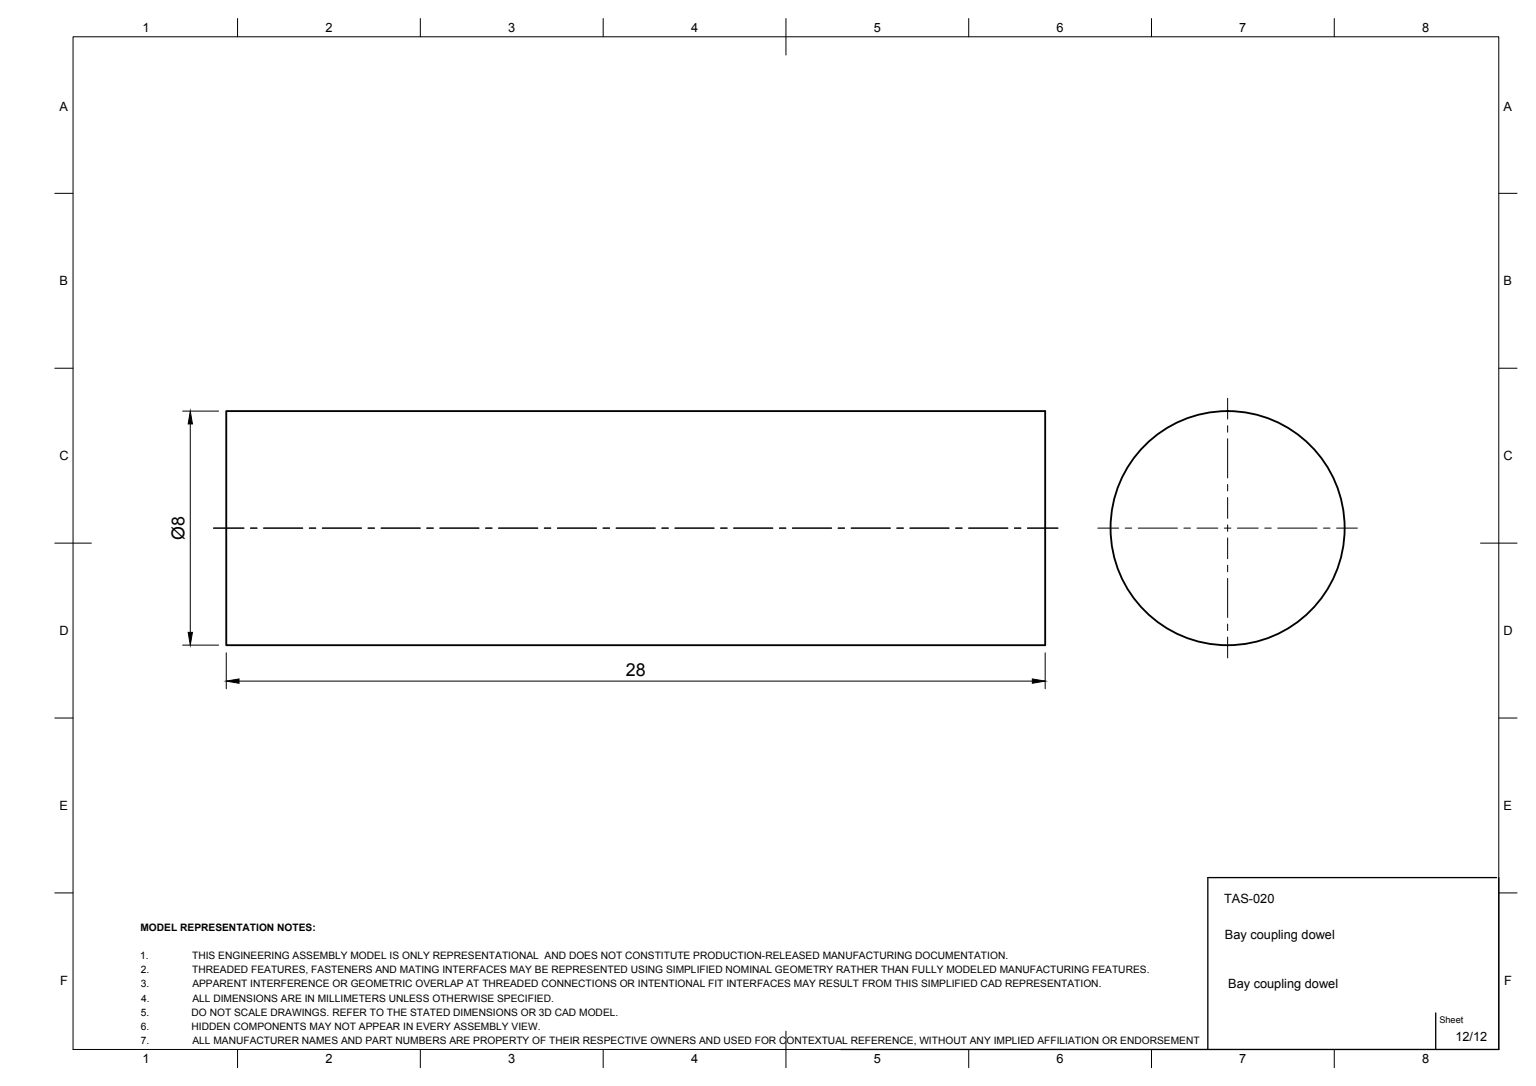
ISO-10303-21;
HEADER;
/* Generated by software containing ST-Developer
 * from STEP Tools, Inc. (www.steptools.com) 
 */

FILE_DESCRIPTION(
/* description */ (''),
/* implementation_level */ '2;1');

FILE_NAME(
/* name */ 'Bay coupling dowel.step',
/* time_stamp */ '2026-11-15T17:46:57-08:00',
/* author */ (''),
/* organization */ (''),
/* preprocessor_version */ 'ST-DEVELOPER v20.2',
/* originating_system */ 'Autodesk Translation Framework v15.17.0.0',
/* authorisation */ '');

FILE_SCHEMA (('AUTOMOTIVE_DESIGN { 1 0 10303 214 3 1 1 }'));
ENDSEC;

DATA;
#10=MECHANICAL_DESIGN_GEOMETRIC_PRESENTATION_REPRESENTATION('',(#386),#12963);
#362=SHAPE_REPRESENTATION_RELATIONSHIP('SRR','None',#13046,#374);
#374=ADVANCED_BREP_SHAPE_REPRESENTATION('',(#398),#12962);
#386=STYLED_ITEM('',(#13115),#398);
#398=MANIFOLD_SOLID_BREP('Body1',#4820);
#570=PLANE('',#5299);
#571=PLANE('',#5300);
#825=FACE_OUTER_BOUND('',#1123,.T.);
#826=FACE_OUTER_BOUND('',#1124,.T.);
#827=FACE_OUTER_BOUND('',#1125,.T.);
#1123=EDGE_LOOP('',(#4426,#4427,#4428,#4429));
#1124=EDGE_LOOP('',(#4430));
#1125=EDGE_LOOP('',(#4431));
#1527=LINE('',#12892,#1929);
#1929=VECTOR('',#6430,0.4);
#2010=CIRCLE('',#5297,0.4);
#2011=CIRCLE('',#5298,0.4);
#2450=VERTEX_POINT('',#12889);
#2451=VERTEX_POINT('',#12891);
#3109=EDGE_CURVE('',#2450,#2450,#2010,.T.);
#3110=EDGE_CURVE('',#2450,#2451,#1527,.T.);
#3111=EDGE_CURVE('',#2451,#2451,#2011,.T.);
#4426=ORIENTED_EDGE('',*,*,#3109,.F.);
#4427=ORIENTED_EDGE('',*,*,#3110,.T.);
#4428=ORIENTED_EDGE('',*,*,#3111,.T.);
#4429=ORIENTED_EDGE('',*,*,#3110,.F.);
#4430=ORIENTED_EDGE('',*,*,#3109,.T.);
#4431=ORIENTED_EDGE('',*,*,#3111,.F.);
#4552=CYLINDRICAL_SURFACE('',#5296,0.4);
#4806=ADVANCED_FACE('',(#825),#4552,.T.);
#4807=ADVANCED_FACE('',(#826),#570,.T.);
#4808=ADVANCED_FACE('',(#827),#571,.F.);
#4820=CLOSED_SHELL('',(#4806,#4807,#4808));
#5295=AXIS2_PLACEMENT_3D('',#12887,#6424,#6425);
#5296=AXIS2_PLACEMENT_3D('',#12888,#6426,#6427);
#5297=AXIS2_PLACEMENT_3D('',#12890,#6428,#6429);
#5298=AXIS2_PLACEMENT_3D('',#12893,#6431,#6432);
#5299=AXIS2_PLACEMENT_3D('',#12894,#6433,#6434);
#5300=AXIS2_PLACEMENT_3D('',#12895,#6435,#6436);
#6424=DIRECTION('axis',(0.,0.,1.));
#6425=DIRECTION('refdir',(1.,0.,0.));
#6426=DIRECTION('center_axis',(0.,0.,1.));
#6427=DIRECTION('ref_axis',(1.,0.,0.));
#6428=DIRECTION('center_axis',(0.,0.,1.));
#6429=DIRECTION('ref_axis',(1.,0.,0.));
#6430=DIRECTION('',(0.,0.,-1.));
#6431=DIRECTION('center_axis',(0.,0.,1.));
#6432=DIRECTION('ref_axis',(1.,0.,0.));
#6433=DIRECTION('center_axis',(0.,0.,1.));
#6434=DIRECTION('ref_axis',(1.,0.,0.));
#6435=DIRECTION('center_axis',(0.,0.,1.));
#6436=DIRECTION('ref_axis',(1.,0.,0.));
#12887=CARTESIAN_POINT('',(0.,0.,0.));
#12888=CARTESIAN_POINT('Origin',(0.,0.,0.));
#12889=CARTESIAN_POINT('',(-0.4,-4.89858719658941E-17,2.8));
#12890=CARTESIAN_POINT('Origin',(0.,0.,2.8));
#12891=CARTESIAN_POINT('',(-0.4,-4.89858719658941E-17,0.));
#12892=CARTESIAN_POINT('',(-0.4,-4.89858719658941E-17,0.));
#12893=CARTESIAN_POINT('Origin',(0.,0.,0.));
#12894=CARTESIAN_POINT('Origin',(0.,0.,2.8));
#12895=CARTESIAN_POINT('Origin',(0.,0.,0.));
#12948=UNCERTAINTY_MEASURE_WITH_UNIT(LENGTH_MEASURE(0.001),#12964,
'DISTANCE_ACCURACY_VALUE',
'Maximum model space distance between geometric entities at asserted c
onnectivities');
#12949=UNCERTAINTY_MEASURE_WITH_UNIT(LENGTH_MEASURE(0.001),#12964,
'DISTANCE_ACCURACY_VALUE',
'Maximum model space distance between geometric entities at asserted c
onnectivities');
#12962=(
GEOMETRIC_REPRESENTATION_CONTEXT(3)
GLOBAL_UNCERTAINTY_ASSIGNED_CONTEXT((#12948))
GLOBAL_UNIT_ASSIGNED_CONTEXT((#12964,#12966,#12967))
REPRESENTATION_CONTEXT('','3D')
);
#12963=(
GEOMETRIC_REPRESENTATION_CONTEXT(3)
GLOBAL_UNCERTAINTY_ASSIGNED_CONTEXT((#12949))
GLOBAL_UNIT_ASSIGNED_CONTEXT((#12964,#12966,#12967))
REPRESENTATION_CONTEXT('','3D')
);
#12964=(
LENGTH_UNIT()
NAMED_UNIT(*)
SI_UNIT(.CENTI.,.METRE.)
);
#12966=(
NAMED_UNIT(*)
PLANE_ANGLE_UNIT()
SI_UNIT($,.RADIAN.)
);
#12967=(
NAMED_UNIT(*)
SI_UNIT($,.STERADIAN.)
SOLID_ANGLE_UNIT()
);
#12980=SHAPE_DEFINITION_REPRESENTATION(#12993,#13046);
#12993=PRODUCT_DEFINITION_SHAPE('',$,#13060);
#13046=SHAPE_REPRESENTATION('',(#5295),#12962);
#13047=PRODUCT_DEFINITION_CONTEXT('part definition',#13088,'design');
#13060=PRODUCT_DEFINITION('Bay coupling dowel','Bay coupling dowel',#13073,
#13047);
#13073=PRODUCT_DEFINITION_FORMATION('',$,#13102);
#13088=APPLICATION_CONTEXT(
'Core Data for Automotive Mechanical Design Process');
#13089=PRODUCT_CONTEXT('part definition',#13088,'mechanical');
#13102=PRODUCT('Bay coupling dowel','Bay coupling dowel',$,(#13089));
#13115=PRESENTATION_STYLE_ASSIGNMENT((#13128));
#13128=SURFACE_STYLE_USAGE(.BOTH.,#13141);
#13141=SURFACE_SIDE_STYLE('',(#13154));
#13154=SURFACE_STYLE_FILL_AREA(#13167);
#13167=FILL_AREA_STYLE('Bay coupling dowel finish',(#13180));
#13180=FILL_AREA_STYLE_COLOUR('Bay coupling dowel finish',#13193);
#13193=COLOUR_RGB('Bay coupling dowel finish',0.43921568627451,0.47843137254902,
0.52156862745098);
ENDSEC;
END-ISO-10303-21;
